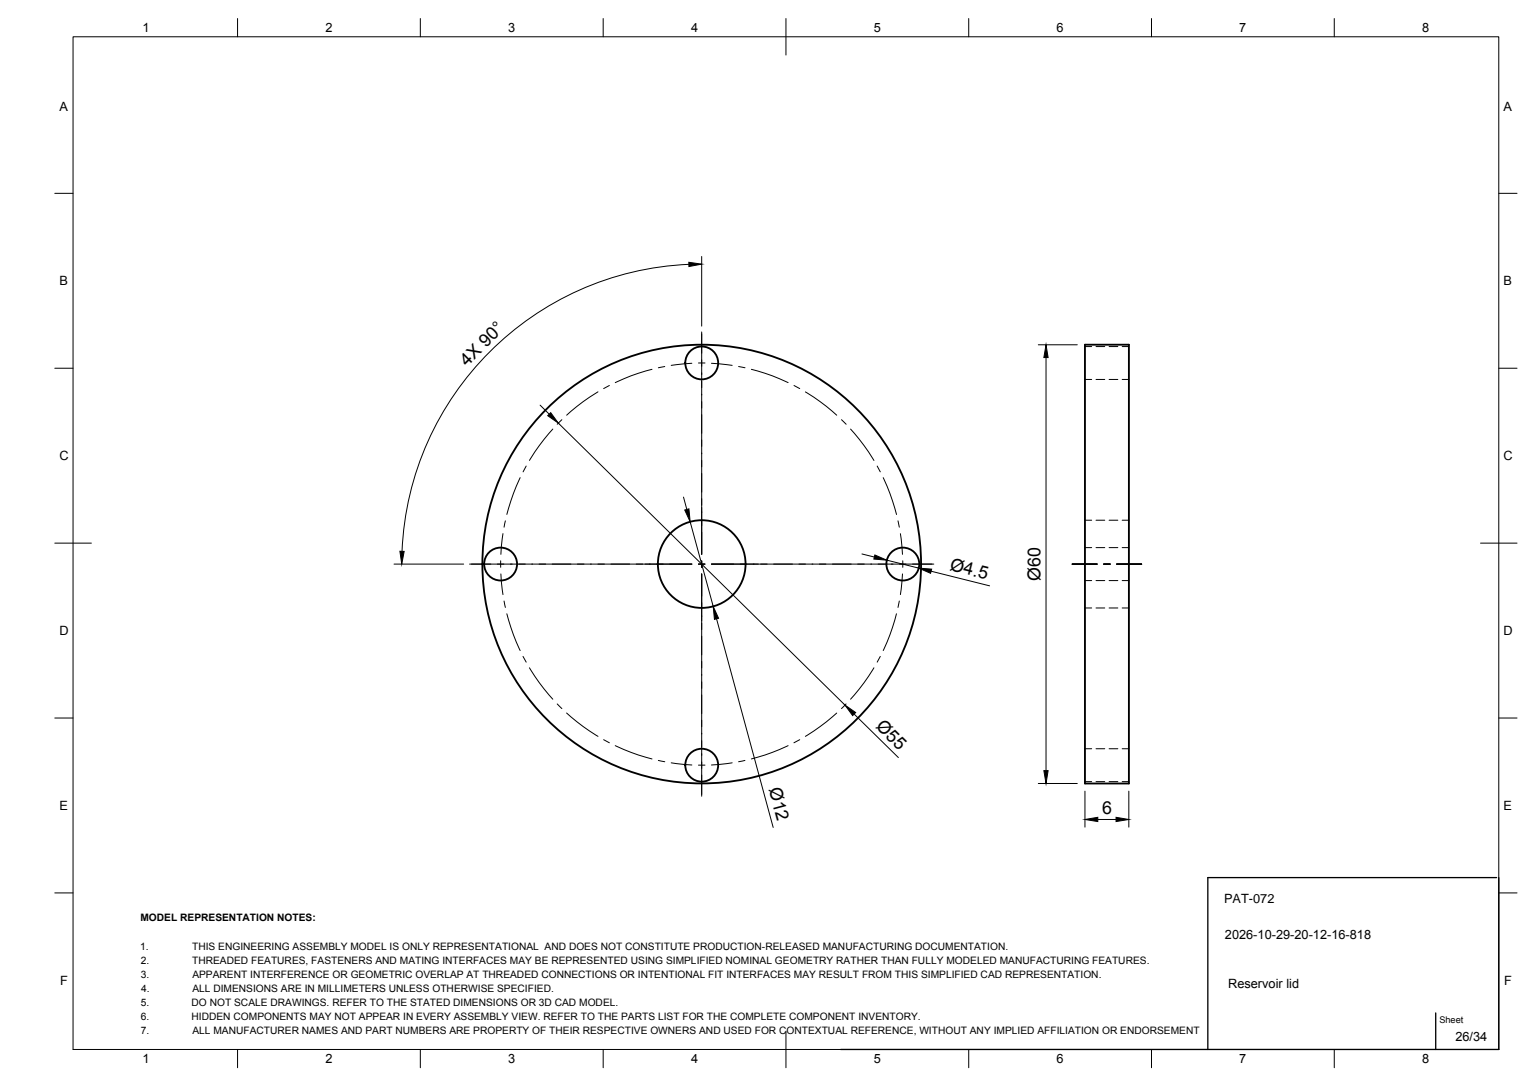
ISO-10303-21;
HEADER;
/* Generated by software containing ST-Developer
 * from STEP Tools, Inc. (www.steptools.com) 
 */

FILE_DESCRIPTION(
/* description */ ('PAT-072'),
/* implementation_level */ '2;1');

FILE_NAME(
/* name */ 'Reservoir lid.step',
/* time_stamp */ '2026-10-29T20:11:56-07:00',
/* author */ (''),
/* organization */ (''),
/* preprocessor_version */ 'ST-DEVELOPER v20.2',
/* originating_system */ 'Autodesk Translation Framework v15.17.0.0',
/* authorisation */ '');

FILE_SCHEMA (('AUTOMOTIVE_DESIGN { 1 0 10303 214 3 1 1 }'));
ENDSEC;

DATA;
#10=MECHANICAL_DESIGN_GEOMETRIC_PRESENTATION_REPRESENTATION('',(#359),#11432);
#287=SHAPE_REPRESENTATION_RELATIONSHIP('SRR','None',#11591,#323);
#323=ADVANCED_BREP_SHAPE_REPRESENTATION('',(#395),#11422);
#359=STYLED_ITEM('',(#11805),#395);
#395=MANIFOLD_SOLID_BREP('Body1',#6094);
#542=FACE_BOUND('',#1590,.T.);
#543=FACE_BOUND('',#1591,.T.);
#544=FACE_BOUND('',#1592,.T.);
#545=FACE_BOUND('',#1593,.T.);
#546=FACE_BOUND('',#1594,.T.);
#547=FACE_BOUND('',#1596,.T.);
#548=FACE_BOUND('',#1597,.T.);
#549=FACE_BOUND('',#1598,.T.);
#550=FACE_BOUND('',#1599,.T.);
#551=FACE_BOUND('',#1600,.T.);
#732=PLANE('',#7064);
#733=PLANE('',#7065);
#1071=FACE_OUTER_BOUND('',#1583,.T.);
#1072=FACE_OUTER_BOUND('',#1584,.T.);
#1073=FACE_OUTER_BOUND('',#1585,.T.);
#1074=FACE_OUTER_BOUND('',#1586,.T.);
#1075=FACE_OUTER_BOUND('',#1587,.T.);
#1076=FACE_OUTER_BOUND('',#1588,.T.);
#1077=FACE_OUTER_BOUND('',#1589,.T.);
#1078=FACE_OUTER_BOUND('',#1595,.T.);
#1583=EDGE_LOOP('',(#5186,#5187,#5188,#5189));
#1584=EDGE_LOOP('',(#5190,#5191,#5192,#5193));
#1585=EDGE_LOOP('',(#5194,#5195,#5196,#5197));
#1586=EDGE_LOOP('',(#5198,#5199,#5200,#5201));
#1587=EDGE_LOOP('',(#5202,#5203,#5204,#5205));
#1588=EDGE_LOOP('',(#5206,#5207,#5208,#5209));
#1589=EDGE_LOOP('',(#5210));
#1590=EDGE_LOOP('',(#5211));
#1591=EDGE_LOOP('',(#5212));
#1592=EDGE_LOOP('',(#5213));
#1593=EDGE_LOOP('',(#5214));
#1594=EDGE_LOOP('',(#5215));
#1595=EDGE_LOOP('',(#5216));
#1596=EDGE_LOOP('',(#5217));
#1597=EDGE_LOOP('',(#5218));
#1598=EDGE_LOOP('',(#5219));
#1599=EDGE_LOOP('',(#5220));
#1600=EDGE_LOOP('',(#5221));
#1998=LINE('',#10896,#2417);
#1999=LINE('',#10902,#2418);
#2000=LINE('',#10908,#2419);
#2001=LINE('',#10914,#2420);
#2002=LINE('',#10920,#2421);
#2003=LINE('',#10926,#2422);
#2417=VECTOR('',#8641,0.6);
#2418=VECTOR('',#8648,0.225);
#2419=VECTOR('',#8655,0.225);
#2420=VECTOR('',#8662,0.225);
#2421=VECTOR('',#8669,0.225);
#2422=VECTOR('',#8676,3.);
#2779=CIRCLE('',#7047,0.6);
#2780=CIRCLE('',#7048,0.6);
#2781=CIRCLE('',#7050,0.225);
#2782=CIRCLE('',#7051,0.225);
#2783=CIRCLE('',#7053,0.225);
#2784=CIRCLE('',#7054,0.225);
#2785=CIRCLE('',#7056,0.225);
#2786=CIRCLE('',#7057,0.225);
#2787=CIRCLE('',#7059,0.225);
#2788=CIRCLE('',#7060,0.225);
#2789=CIRCLE('',#7062,3.);
#2790=CIRCLE('',#7063,3.);
#3202=VERTEX_POINT('',#10893);
#3203=VERTEX_POINT('',#10895);
#3204=VERTEX_POINT('',#10899);
#3205=VERTEX_POINT('',#10901);
#3206=VERTEX_POINT('',#10905);
#3207=VERTEX_POINT('',#10907);
#3208=VERTEX_POINT('',#10911);
#3209=VERTEX_POINT('',#10913);
#3210=VERTEX_POINT('',#10917);
#3211=VERTEX_POINT('',#10919);
#3212=VERTEX_POINT('',#10923);
#3213=VERTEX_POINT('',#10925);
#3882=EDGE_CURVE('',#3202,#3202,#2779,.T.);
#3883=EDGE_CURVE('',#3202,#3203,#1998,.T.);
#3884=EDGE_CURVE('',#3203,#3203,#2780,.T.);
#3885=EDGE_CURVE('',#3204,#3204,#2781,.T.);
#3886=EDGE_CURVE('',#3204,#3205,#1999,.T.);
#3887=EDGE_CURVE('',#3205,#3205,#2782,.T.);
#3888=EDGE_CURVE('',#3206,#3206,#2783,.T.);
#3889=EDGE_CURVE('',#3206,#3207,#2000,.T.);
#3890=EDGE_CURVE('',#3207,#3207,#2784,.T.);
#3891=EDGE_CURVE('',#3208,#3208,#2785,.T.);
#3892=EDGE_CURVE('',#3208,#3209,#2001,.T.);
#3893=EDGE_CURVE('',#3209,#3209,#2786,.T.);
#3894=EDGE_CURVE('',#3210,#3210,#2787,.T.);
#3895=EDGE_CURVE('',#3210,#3211,#2002,.T.);
#3896=EDGE_CURVE('',#3211,#3211,#2788,.T.);
#3897=EDGE_CURVE('',#3212,#3212,#2789,.T.);
#3898=EDGE_CURVE('',#3212,#3213,#2003,.T.);
#3899=EDGE_CURVE('',#3213,#3213,#2790,.T.);
#5186=ORIENTED_EDGE('',*,*,#3882,.F.);
#5187=ORIENTED_EDGE('',*,*,#3883,.T.);
#5188=ORIENTED_EDGE('',*,*,#3884,.F.);
#5189=ORIENTED_EDGE('',*,*,#3883,.F.);
#5190=ORIENTED_EDGE('',*,*,#3885,.F.);
#5191=ORIENTED_EDGE('',*,*,#3886,.T.);
#5192=ORIENTED_EDGE('',*,*,#3887,.F.);
#5193=ORIENTED_EDGE('',*,*,#3886,.F.);
#5194=ORIENTED_EDGE('',*,*,#3888,.F.);
#5195=ORIENTED_EDGE('',*,*,#3889,.T.);
#5196=ORIENTED_EDGE('',*,*,#3890,.F.);
#5197=ORIENTED_EDGE('',*,*,#3889,.F.);
#5198=ORIENTED_EDGE('',*,*,#3891,.F.);
#5199=ORIENTED_EDGE('',*,*,#3892,.T.);
#5200=ORIENTED_EDGE('',*,*,#3893,.F.);
#5201=ORIENTED_EDGE('',*,*,#3892,.F.);
#5202=ORIENTED_EDGE('',*,*,#3894,.F.);
#5203=ORIENTED_EDGE('',*,*,#3895,.T.);
#5204=ORIENTED_EDGE('',*,*,#3896,.F.);
#5205=ORIENTED_EDGE('',*,*,#3895,.F.);
#5206=ORIENTED_EDGE('',*,*,#3897,.F.);
#5207=ORIENTED_EDGE('',*,*,#3898,.T.);
#5208=ORIENTED_EDGE('',*,*,#3899,.T.);
#5209=ORIENTED_EDGE('',*,*,#3898,.F.);
#5210=ORIENTED_EDGE('',*,*,#3897,.T.);
#5211=ORIENTED_EDGE('',*,*,#3884,.T.);
#5212=ORIENTED_EDGE('',*,*,#3887,.T.);
#5213=ORIENTED_EDGE('',*,*,#3890,.T.);
#5214=ORIENTED_EDGE('',*,*,#3893,.T.);
#5215=ORIENTED_EDGE('',*,*,#3896,.T.);
#5216=ORIENTED_EDGE('',*,*,#3899,.F.);
#5217=ORIENTED_EDGE('',*,*,#3882,.T.);
#5218=ORIENTED_EDGE('',*,*,#3885,.T.);
#5219=ORIENTED_EDGE('',*,*,#3888,.T.);
#5220=ORIENTED_EDGE('',*,*,#3891,.T.);
#5221=ORIENTED_EDGE('',*,*,#3894,.T.);
#5671=CYLINDRICAL_SURFACE('',#7046,0.6);
#5672=CYLINDRICAL_SURFACE('',#7049,0.225);
#5673=CYLINDRICAL_SURFACE('',#7052,0.225);
#5674=CYLINDRICAL_SURFACE('',#7055,0.225);
#5675=CYLINDRICAL_SURFACE('',#7058,0.225);
#5676=CYLINDRICAL_SURFACE('',#7061,3.);
#5970=ADVANCED_FACE('',(#1071),#5671,.F.);
#5971=ADVANCED_FACE('',(#1072),#5672,.F.);
#5972=ADVANCED_FACE('',(#1073),#5673,.F.);
#5973=ADVANCED_FACE('',(#1074),#5674,.F.);
#5974=ADVANCED_FACE('',(#1075),#5675,.F.);
#5975=ADVANCED_FACE('',(#1076),#5676,.T.);
#5976=ADVANCED_FACE('',(#1077,#542,#543,#544,#545,#546),#732,.T.);
#5977=ADVANCED_FACE('',(#1078,#547,#548,#549,#550,#551),#733,.F.);
#6094=CLOSED_SHELL('',(#5970,#5971,#5972,#5973,#5974,#5975,#5976,#5977));
#7045=AXIS2_PLACEMENT_3D('',#10891,#8635,#8636);
#7046=AXIS2_PLACEMENT_3D('',#10892,#8637,#8638);
#7047=AXIS2_PLACEMENT_3D('',#10894,#8639,#8640);
#7048=AXIS2_PLACEMENT_3D('',#10897,#8642,#8643);
#7049=AXIS2_PLACEMENT_3D('',#10898,#8644,#8645);
#7050=AXIS2_PLACEMENT_3D('',#10900,#8646,#8647);
#7051=AXIS2_PLACEMENT_3D('',#10903,#8649,#8650);
#7052=AXIS2_PLACEMENT_3D('',#10904,#8651,#8652);
#7053=AXIS2_PLACEMENT_3D('',#10906,#8653,#8654);
#7054=AXIS2_PLACEMENT_3D('',#10909,#8656,#8657);
#7055=AXIS2_PLACEMENT_3D('',#10910,#8658,#8659);
#7056=AXIS2_PLACEMENT_3D('',#10912,#8660,#8661);
#7057=AXIS2_PLACEMENT_3D('',#10915,#8663,#8664);
#7058=AXIS2_PLACEMENT_3D('',#10916,#8665,#8666);
#7059=AXIS2_PLACEMENT_3D('',#10918,#8667,#8668);
#7060=AXIS2_PLACEMENT_3D('',#10921,#8670,#8671);
#7061=AXIS2_PLACEMENT_3D('',#10922,#8672,#8673);
#7062=AXIS2_PLACEMENT_3D('',#10924,#8674,#8675);
#7063=AXIS2_PLACEMENT_3D('',#10927,#8677,#8678);
#7064=AXIS2_PLACEMENT_3D('',#10928,#8679,#8680);
#7065=AXIS2_PLACEMENT_3D('',#10929,#8681,#8682);
#8635=DIRECTION('axis',(0.,0.,1.));
#8636=DIRECTION('refdir',(1.,0.,0.));
#8637=DIRECTION('center_axis',(0.,0.,1.));
#8638=DIRECTION('ref_axis',(1.,0.,0.));
#8639=DIRECTION('center_axis',(0.,0.,1.));
#8640=DIRECTION('ref_axis',(1.,0.,0.));
#8641=DIRECTION('',(0.,0.,1.));
#8642=DIRECTION('center_axis',(0.,0.,-1.));
#8643=DIRECTION('ref_axis',(1.,0.,0.));
#8644=DIRECTION('center_axis',(0.,0.,1.));
#8645=DIRECTION('ref_axis',(1.,0.,0.));
#8646=DIRECTION('center_axis',(0.,0.,1.));
#8647=DIRECTION('ref_axis',(1.,0.,0.));
#8648=DIRECTION('',(0.,0.,1.));
#8649=DIRECTION('center_axis',(0.,0.,-1.));
#8650=DIRECTION('ref_axis',(1.,0.,0.));
#8651=DIRECTION('center_axis',(0.,0.,1.));
#8652=DIRECTION('ref_axis',(1.,0.,0.));
#8653=DIRECTION('center_axis',(0.,0.,1.));
#8654=DIRECTION('ref_axis',(1.,0.,0.));
#8655=DIRECTION('',(0.,0.,1.));
#8656=DIRECTION('center_axis',(0.,0.,-1.));
#8657=DIRECTION('ref_axis',(1.,0.,0.));
#8658=DIRECTION('center_axis',(0.,0.,1.));
#8659=DIRECTION('ref_axis',(1.,0.,0.));
#8660=DIRECTION('center_axis',(0.,0.,1.));
#8661=DIRECTION('ref_axis',(1.,0.,0.));
#8662=DIRECTION('',(0.,0.,1.));
#8663=DIRECTION('center_axis',(0.,0.,-1.));
#8664=DIRECTION('ref_axis',(1.,0.,0.));
#8665=DIRECTION('center_axis',(0.,0.,1.));
#8666=DIRECTION('ref_axis',(1.,0.,0.));
#8667=DIRECTION('center_axis',(0.,0.,1.));
#8668=DIRECTION('ref_axis',(1.,0.,0.));
#8669=DIRECTION('',(0.,0.,1.));
#8670=DIRECTION('center_axis',(0.,0.,-1.));
#8671=DIRECTION('ref_axis',(1.,0.,0.));
#8672=DIRECTION('center_axis',(0.,0.,1.));
#8673=DIRECTION('ref_axis',(1.,0.,0.));
#8674=DIRECTION('center_axis',(0.,0.,1.));
#8675=DIRECTION('ref_axis',(1.,0.,0.));
#8676=DIRECTION('',(0.,0.,-1.));
#8677=DIRECTION('center_axis',(0.,0.,1.));
#8678=DIRECTION('ref_axis',(1.,0.,0.));
#8679=DIRECTION('center_axis',(0.,0.,1.));
#8680=DIRECTION('ref_axis',(1.,0.,0.));
#8681=DIRECTION('center_axis',(0.,0.,1.));
#8682=DIRECTION('ref_axis',(1.,0.,0.));
#10891=CARTESIAN_POINT('',(0.,0.,0.));
#10892=CARTESIAN_POINT('Origin',(0.,0.,15.));
#10893=CARTESIAN_POINT('',(-0.6,-7.34788079488412E-17,15.1));
#10894=CARTESIAN_POINT('Origin',(0.,0.,15.1));
#10895=CARTESIAN_POINT('',(-0.6,7.34788079488412E-17,15.7));
#10896=CARTESIAN_POINT('',(-0.6,-7.34788079488412E-17,15.));
#10897=CARTESIAN_POINT('Origin',(0.,0.,15.7));
#10898=CARTESIAN_POINT('Origin',(-2.75,3.36777869765522E-16,14.9));
#10899=CARTESIAN_POINT('',(-2.975,3.09223316784707E-16,15.1));
#10900=CARTESIAN_POINT('Origin',(-2.75,3.36777869765522E-16,15.1));
#10901=CARTESIAN_POINT('',(-2.975,3.64332422746338E-16,15.7));
#10902=CARTESIAN_POINT('',(-2.975,3.09223316784707E-16,14.9));
#10903=CARTESIAN_POINT('Origin',(-2.75,3.36777869765522E-16,15.7));
#10904=CARTESIAN_POINT('Origin',(1.68388934882761E-16,2.75,14.9));
#10905=CARTESIAN_POINT('',(-0.225,2.75,15.1));
#10906=CARTESIAN_POINT('Origin',(1.68388934882761E-16,2.75,15.1));
#10907=CARTESIAN_POINT('',(-0.225,2.75,15.7));
#10908=CARTESIAN_POINT('',(-0.225,2.75,14.9));
#10909=CARTESIAN_POINT('Origin',(1.68388934882761E-16,2.75,15.7));
#10910=CARTESIAN_POINT('Origin',(2.75,0.,14.9));
#10911=CARTESIAN_POINT('',(2.525,-2.75545529808155E-17,15.1));
#10912=CARTESIAN_POINT('Origin',(2.75,0.,15.1));
#10913=CARTESIAN_POINT('',(2.525,2.75545529808155E-17,15.7));
#10914=CARTESIAN_POINT('',(2.525,-2.75545529808155E-17,14.9));
#10915=CARTESIAN_POINT('Origin',(2.75,0.,15.7));
#10916=CARTESIAN_POINT('Origin',(-5.05166804648283E-16,-2.75,14.9));
#10917=CARTESIAN_POINT('',(-0.225000000000001,-2.75,15.1));
#10918=CARTESIAN_POINT('Origin',(-5.05166804648283E-16,-2.75,15.1));
#10919=CARTESIAN_POINT('',(-0.225000000000001,-2.75,15.7));
#10920=CARTESIAN_POINT('',(-0.225000000000001,-2.75,14.9));
#10921=CARTESIAN_POINT('Origin',(-5.05166804648283E-16,-2.75,15.7));
#10922=CARTESIAN_POINT('Origin',(0.,0.,15.1));
#10923=CARTESIAN_POINT('',(-3.,-3.67394039744206E-16,15.7));
#10924=CARTESIAN_POINT('Origin',(0.,0.,15.7));
#10925=CARTESIAN_POINT('',(-3.,-3.67394039744206E-16,15.1));
#10926=CARTESIAN_POINT('',(-3.,-3.67394039744206E-16,15.1));
#10927=CARTESIAN_POINT('Origin',(0.,0.,15.1));
#10928=CARTESIAN_POINT('Origin',(0.,0.,15.7));
#10929=CARTESIAN_POINT('Origin',(0.,0.,15.1));
#11383=UNCERTAINTY_MEASURE_WITH_UNIT(LENGTH_MEASURE(0.001),#11433,
'DISTANCE_ACCURACY_VALUE',
'Maximum model space distance between geometric entities at asserted c
onnectivities');
#11393=UNCERTAINTY_MEASURE_WITH_UNIT(LENGTH_MEASURE(0.001),#11433,
'DISTANCE_ACCURACY_VALUE',
'Maximum model space distance between geometric entities at asserted c
onnectivities');
#11422=(
GEOMETRIC_REPRESENTATION_CONTEXT(3)
GLOBAL_UNCERTAINTY_ASSIGNED_CONTEXT((#11383))
GLOBAL_UNIT_ASSIGNED_CONTEXT((#11433,#11435,#11436))
REPRESENTATION_CONTEXT('','3D')
);
#11432=(
GEOMETRIC_REPRESENTATION_CONTEXT(3)
GLOBAL_UNCERTAINTY_ASSIGNED_CONTEXT((#11393))
GLOBAL_UNIT_ASSIGNED_CONTEXT((#11433,#11435,#11436))
REPRESENTATION_CONTEXT('','3D')
);
#11433=(
LENGTH_UNIT()
NAMED_UNIT(*)
SI_UNIT(.CENTI.,.METRE.)
);
#11435=(
NAMED_UNIT(*)
PLANE_ANGLE_UNIT()
SI_UNIT($,.RADIAN.)
);
#11436=(
NAMED_UNIT(*)
SI_UNIT($,.STERADIAN.)
SOLID_ANGLE_UNIT()
);
#11465=SHAPE_DEFINITION_REPRESENTATION(#11503,#11591);
#11503=PRODUCT_DEFINITION_SHAPE('',$,#11630);
#11591=SHAPE_REPRESENTATION('',(#7045),#11422);
#11601=PRODUCT_DEFINITION_CONTEXT('part definition',#11717,'design');
#11630=PRODUCT_DEFINITION('Reservoir lid','Reservoir lid',#11668,
#11601);
#11668=PRODUCT_DEFINITION_FORMATION('',$,#11747);
#11717=APPLICATION_CONTEXT(
'Core Data for Automotive Mechanical Design Process');
#11718=PRODUCT_CONTEXT('part definition',#11717,'mechanical');
#11747=PRODUCT('Reservoir lid','Reservoir lid',
'Reservoir lid',(#11718));
#11799=COLOUR_RGB('Light Blue',0.38,0.62,0.78);
#11800=FILL_AREA_STYLE_COLOUR('',#11799);
#11801=FILL_AREA_STYLE('',(#11800));
#11802=SURFACE_STYLE_FILL_AREA(#11801);
#11803=SURFACE_SIDE_STYLE('',(#11802));
#11804=SURFACE_STYLE_USAGE(.BOTH.,#11803);
#11805=PRESENTATION_STYLE_ASSIGNMENT((#11804));
ENDSEC;
END-ISO-10303-21;
